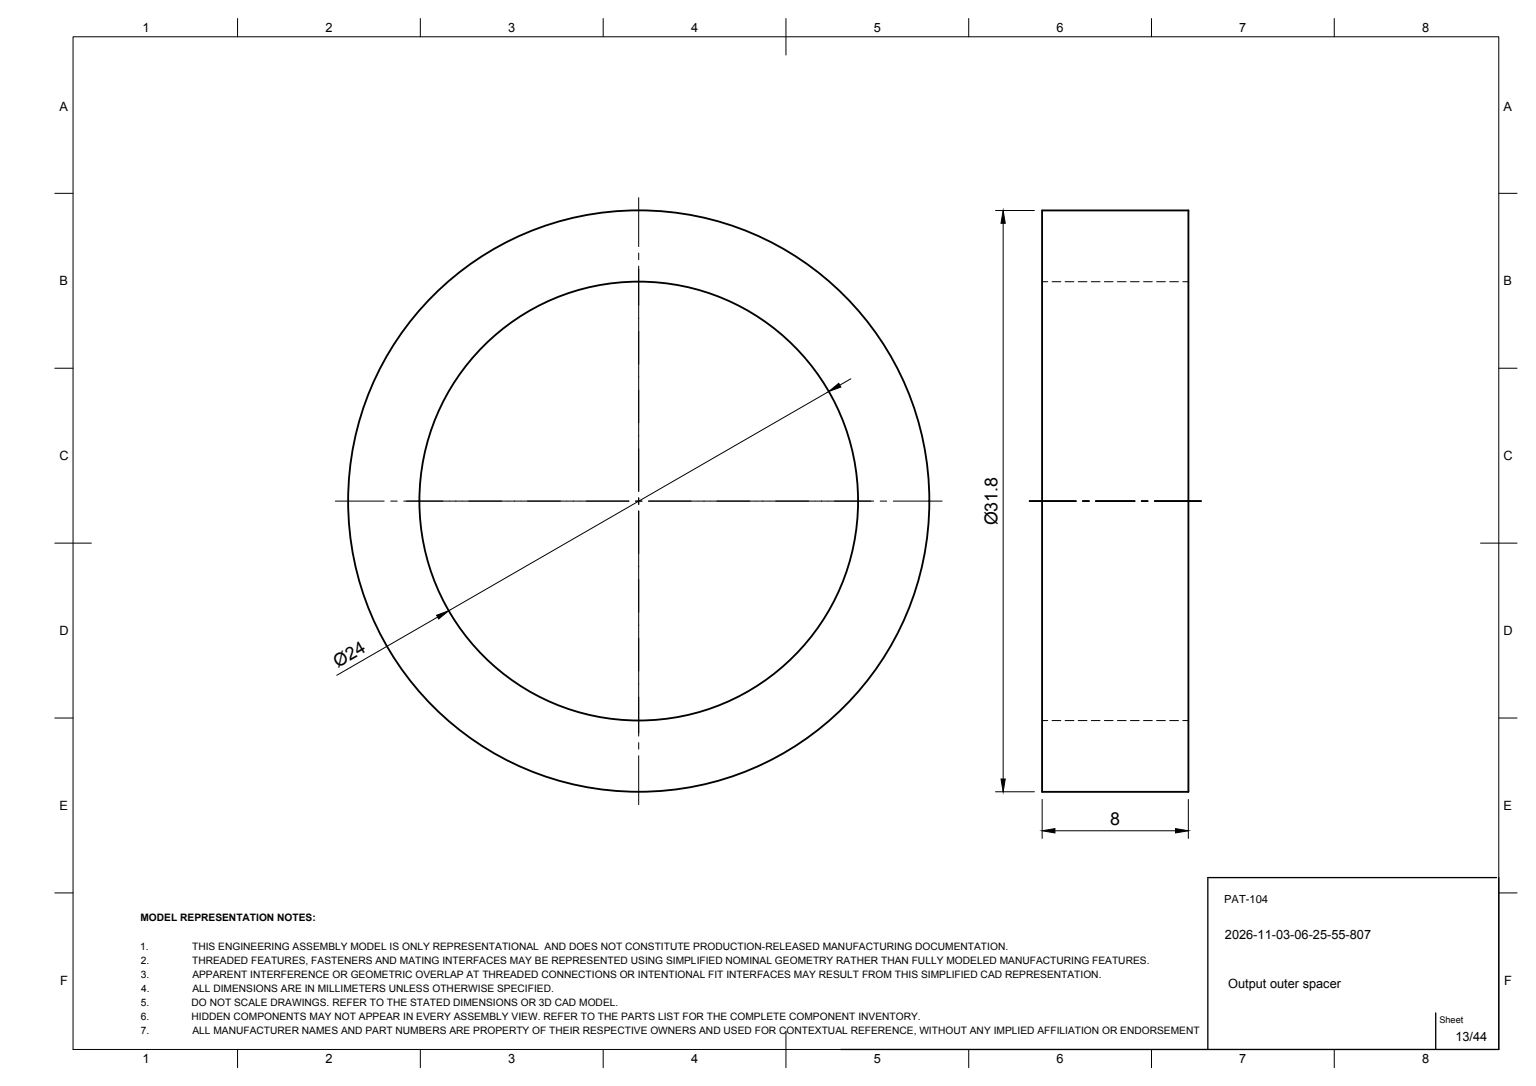
ISO-10303-21;
HEADER;
/* Generated by software containing ST-Developer
 * from STEP Tools, Inc. (www.steptools.com) 
 */

FILE_DESCRIPTION(
/* description */ ('Timing belt drive module 2 mm Pitch Timing 20T-40T'),

/* implementation_level */ '2;1');

FILE_NAME(
/* name */ 'Output outer spacer.step',
/* time_stamp */ '2026-10-28T03:25:12-07:00',
/* author */ (''),
/* organization */ (''),
/* preprocessor_version */ 'ST-DEVELOPER v20.2',
/* originating_system */ 'Autodesk Translation Framework v15.17.0.0',
/* authorisation */ '');

FILE_SCHEMA (('AUTOMOTIVE_DESIGN { 1 0 10303 214 3 1 1 }'));
ENDSEC;

DATA;
#10=MECHANICAL_DESIGN_GEOMETRIC_PRESENTATION_REPRESENTATION('',(#536),#17830);
#450=SHAPE_REPRESENTATION_RELATIONSHIP('SRR','None',#18020,#493);
#493=ADVANCED_BREP_SHAPE_REPRESENTATION('',(#594),#17795);
#536=STYLED_ITEM('',(#18331),#594);
#594=MANIFOLD_SOLID_BREP('Body1',#8993);
#699=FACE_BOUND('',#1674,.T.);
#700=FACE_BOUND('',#1676,.T.);
#839=PLANE('',#9787);
#840=PLANE('',#9788);
#1088=FACE_OUTER_BOUND('',#1671,.T.);
#1089=FACE_OUTER_BOUND('',#1672,.T.);
#1090=FACE_OUTER_BOUND('',#1673,.T.);
#1091=FACE_OUTER_BOUND('',#1675,.T.);
#1671=EDGE_LOOP('',(#6361,#6362,#6363,#6364));
#1672=EDGE_LOOP('',(#6365,#6366,#6367,#6368));
#1673=EDGE_LOOP('',(#6369));
#1674=EDGE_LOOP('',(#6370));
#1675=EDGE_LOOP('',(#6371));
#1676=EDGE_LOOP('',(#6372));
#2264=CIRCLE('',#9782,1.2);
#2265=CIRCLE('',#9783,1.2);
#2266=CIRCLE('',#9785,1.59);
#2267=CIRCLE('',#9786,1.59);
#2960=LINE('',#14508,#3438);
#2961=LINE('',#14514,#3439);
#3438=VECTOR('',#11513,1.2);
#3439=VECTOR('',#11520,1.59);
#3942=VERTEX_POINT('',#14505);
#3943=VERTEX_POINT('',#14507);
#3944=VERTEX_POINT('',#14511);
#3945=VERTEX_POINT('',#14513);
#4863=EDGE_CURVE('',#3942,#3942,#2264,.T.);
#4864=EDGE_CURVE('',#3942,#3943,#2960,.T.);
#4865=EDGE_CURVE('',#3943,#3943,#2265,.T.);
#4866=EDGE_CURVE('',#3944,#3944,#2266,.T.);
#4867=EDGE_CURVE('',#3944,#3945,#2961,.T.);
#4868=EDGE_CURVE('',#3945,#3945,#2267,.T.);
#6361=ORIENTED_EDGE('',*,*,#4863,.F.);
#6362=ORIENTED_EDGE('',*,*,#4864,.T.);
#6363=ORIENTED_EDGE('',*,*,#4865,.T.);
#6364=ORIENTED_EDGE('',*,*,#4864,.F.);
#6365=ORIENTED_EDGE('',*,*,#4866,.F.);
#6366=ORIENTED_EDGE('',*,*,#4867,.T.);
#6367=ORIENTED_EDGE('',*,*,#4868,.T.);
#6368=ORIENTED_EDGE('',*,*,#4867,.F.);
#6369=ORIENTED_EDGE('',*,*,#4866,.T.);
#6370=ORIENTED_EDGE('',*,*,#4863,.T.);
#6371=ORIENTED_EDGE('',*,*,#4868,.F.);
#6372=ORIENTED_EDGE('',*,*,#4865,.F.);
#8241=CYLINDRICAL_SURFACE('',#9781,1.2);
#8242=CYLINDRICAL_SURFACE('',#9784,1.59);
#8586=ADVANCED_FACE('',(#1088),#8241,.F.);
#8587=ADVANCED_FACE('',(#1089),#8242,.T.);
#8588=ADVANCED_FACE('',(#1090,#699),#839,.T.);
#8589=ADVANCED_FACE('',(#1091,#700),#840,.F.);
#8993=CLOSED_SHELL('',(#8586,#8587,#8588,#8589));
#9780=AXIS2_PLACEMENT_3D('',#14503,#11507,#11508);
#9781=AXIS2_PLACEMENT_3D('',#14504,#11509,#11510);
#9782=AXIS2_PLACEMENT_3D('',#14506,#11511,#11512);
#9783=AXIS2_PLACEMENT_3D('',#14509,#11514,#11515);
#9784=AXIS2_PLACEMENT_3D('',#14510,#11516,#11517);
#9785=AXIS2_PLACEMENT_3D('',#14512,#11518,#11519);
#9786=AXIS2_PLACEMENT_3D('',#14515,#11521,#11522);
#9787=AXIS2_PLACEMENT_3D('',#14516,#11523,#11524);
#9788=AXIS2_PLACEMENT_3D('',#14517,#11525,#11526);
#11507=DIRECTION('axis',(0.,0.,1.));
#11508=DIRECTION('refdir',(1.,0.,0.));
#11509=DIRECTION('center_axis',(0.,1.,0.));
#11510=DIRECTION('ref_axis',(1.,0.,0.));
#11511=DIRECTION('center_axis',(0.,-1.,0.));
#11512=DIRECTION('ref_axis',(1.,0.,0.));
#11513=DIRECTION('',(0.,-1.,0.));
#11514=DIRECTION('center_axis',(0.,-1.,0.));
#11515=DIRECTION('ref_axis',(1.,0.,0.));
#11516=DIRECTION('center_axis',(0.,1.,0.));
#11517=DIRECTION('ref_axis',(1.,0.,0.));
#11518=DIRECTION('center_axis',(0.,1.,0.));
#11519=DIRECTION('ref_axis',(1.,0.,0.));
#11520=DIRECTION('',(0.,-1.,0.));
#11521=DIRECTION('center_axis',(0.,1.,0.));
#11522=DIRECTION('ref_axis',(1.,0.,0.));
#11523=DIRECTION('center_axis',(0.,1.,0.));
#11524=DIRECTION('ref_axis',(1.,0.,0.));
#11525=DIRECTION('center_axis',(0.,1.,0.));
#11526=DIRECTION('ref_axis',(1.,0.,0.));
#14503=CARTESIAN_POINT('',(0.,0.,0.));
#14504=CARTESIAN_POINT('Origin',(6.97091003018116,-0.4,7.));
#14505=CARTESIAN_POINT('',(5.77091003018116,0.4,7.));
#14506=CARTESIAN_POINT('Origin',(6.97091003018116,0.4,7.));
#14507=CARTESIAN_POINT('',(5.77091003018116,-0.4,7.));
#14508=CARTESIAN_POINT('',(5.77091003018116,-0.4,7.));
#14509=CARTESIAN_POINT('Origin',(6.97091003018116,-0.4,7.));
#14510=CARTESIAN_POINT('Origin',(6.97091003018116,-0.4,7.));
#14511=CARTESIAN_POINT('',(5.38091003018116,0.4,7.));
#14512=CARTESIAN_POINT('Origin',(6.97091003018116,0.4,7.));
#14513=CARTESIAN_POINT('',(5.38091003018116,-0.4,7.));
#14514=CARTESIAN_POINT('',(5.38091003018116,-0.4,7.));
#14515=CARTESIAN_POINT('Origin',(6.97091003018116,-0.4,7.));
#14516=CARTESIAN_POINT('Origin',(6.97091003018116,0.4,7.));
#14517=CARTESIAN_POINT('Origin',(6.97091003018116,-0.4,7.));
#17745=UNCERTAINTY_MEASURE_WITH_UNIT(LENGTH_MEASURE(0.001),#17831,
'DISTANCE_ACCURACY_VALUE',
'Maximum model space distance between geometric entities at asserted c
onnectivities');
#17780=UNCERTAINTY_MEASURE_WITH_UNIT(LENGTH_MEASURE(0.001),#17831,
'DISTANCE_ACCURACY_VALUE',
'Maximum model space distance between geometric entities at asserted c
onnectivities');
#17795=(
GEOMETRIC_REPRESENTATION_CONTEXT(3)
GLOBAL_UNCERTAINTY_ASSIGNED_CONTEXT((#17745))
GLOBAL_UNIT_ASSIGNED_CONTEXT((#17831,#17833,#17834))
REPRESENTATION_CONTEXT('','3D')
);
#17830=(
GEOMETRIC_REPRESENTATION_CONTEXT(3)
GLOBAL_UNCERTAINTY_ASSIGNED_CONTEXT((#17780))
GLOBAL_UNIT_ASSIGNED_CONTEXT((#17831,#17833,#17834))
REPRESENTATION_CONTEXT('','3D')
);
#17831=(
LENGTH_UNIT()
NAMED_UNIT(*)
SI_UNIT(.CENTI.,.METRE.)
);
#17833=(
NAMED_UNIT(*)
PLANE_ANGLE_UNIT()
SI_UNIT($,.RADIAN.)
);
#17834=(
NAMED_UNIT(*)
SI_UNIT($,.STERADIAN.)
SOLID_ANGLE_UNIT()
);
#17849=SHAPE_DEFINITION_REPRESENTATION(#17898,#18020);
#17898=PRODUCT_DEFINITION_SHAPE('',$,#18070);
#18020=SHAPE_REPRESENTATION('',(#9780),#17795);
#18055=PRODUCT_DEFINITION_CONTEXT('part definition',#18204,'design');
#18070=PRODUCT_DEFINITION('Output outer spacer','Output outer spacer',#18119,
#18055);
#18119=PRODUCT_DEFINITION_FORMATION('',$,#18220);
#18204=APPLICATION_CONTEXT(
'Core Data for Automotive Mechanical Design Process');
#18205=PRODUCT_CONTEXT('part definition',#18204,'mechanical');
#18220=PRODUCT('Output outer spacer','Output outer spacer',
'Output outer spacer',(#18205));
#18325=COLOUR_RGB('Off White',0.89,0.88,0.83);
#18326=FILL_AREA_STYLE_COLOUR('',#18325);
#18327=FILL_AREA_STYLE('',(#18326));
#18328=SURFACE_STYLE_FILL_AREA(#18327);
#18329=SURFACE_SIDE_STYLE('',(#18328));
#18330=SURFACE_STYLE_USAGE(.BOTH.,#18329);
#18331=PRESENTATION_STYLE_ASSIGNMENT((#18330));
ENDSEC;
END-ISO-10303-21;
